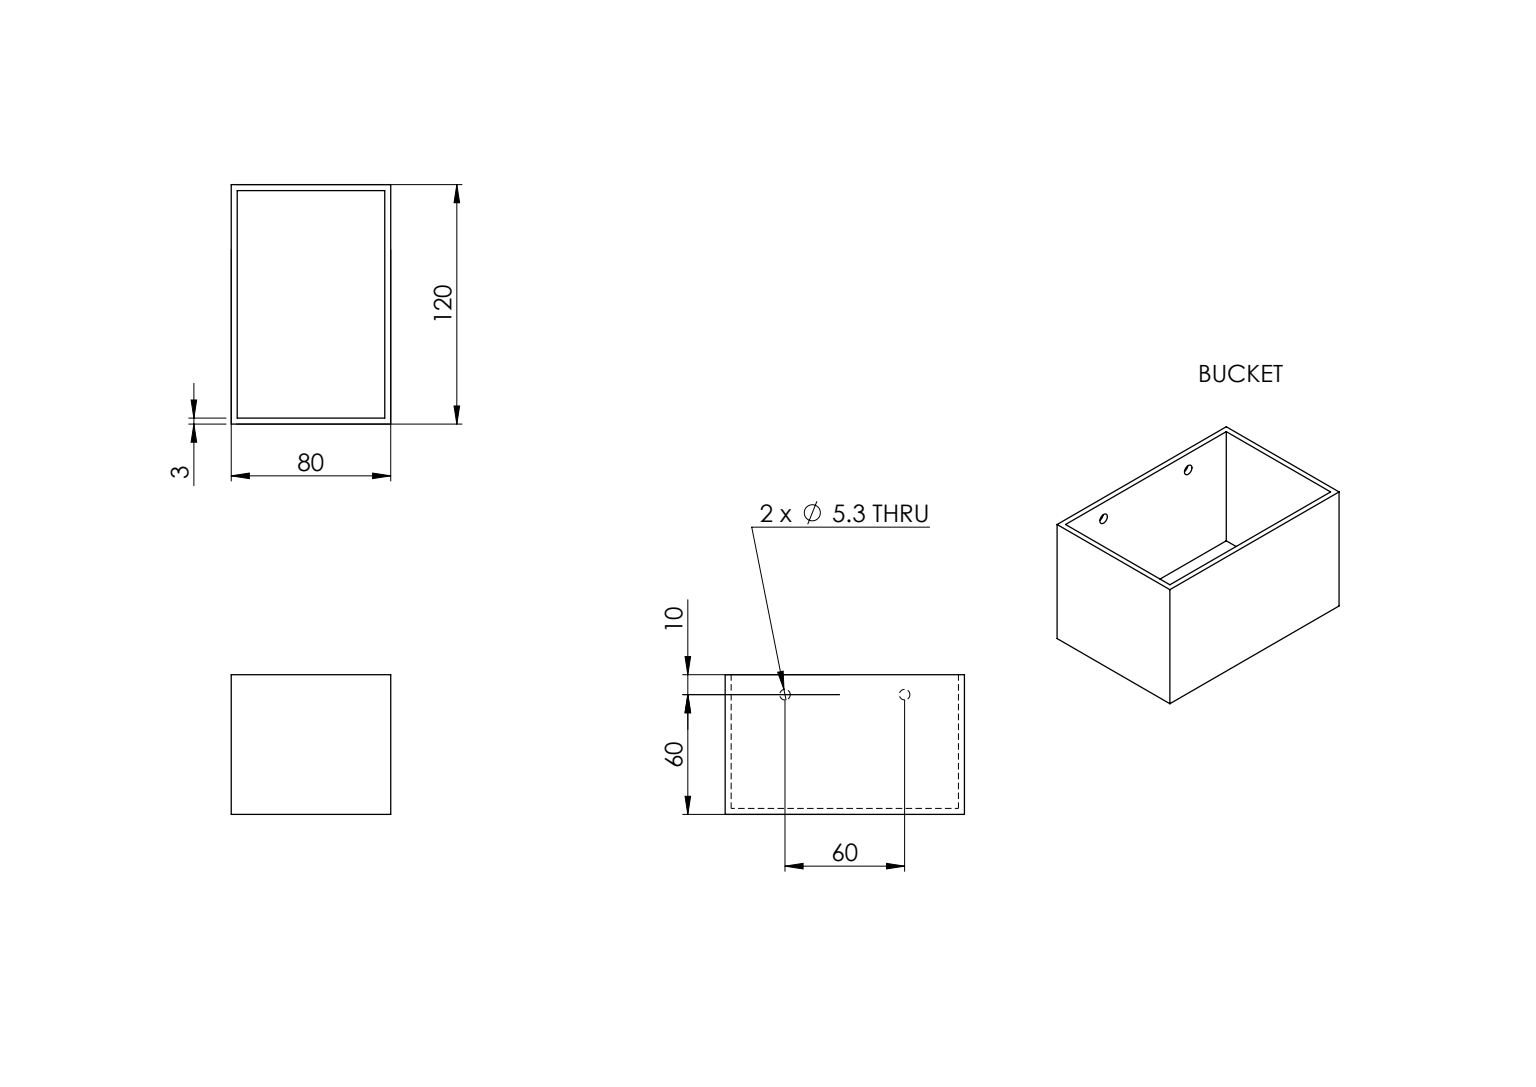
ISO-10303-21;
HEADER;
FILE_DESCRIPTION (('STEP AP214'),
    '1' );
FILE_NAME ('bucket.step',
    '2026-10-31T03:46:07',
    ( '' ),
    ( '' ),
    'SwSTEP 2.0',
    'SolidWorks 2026',
    '' );
FILE_SCHEMA (( 'AUTOMOTIVE_DESIGN' ));
ENDSEC;

DATA;
#88=ADVANCED_FACE ( 'NONE', ( #16201 ), #18340, .T. ) ;
#110=SHAPE_DEFINITION_REPRESENTATION ( #7281, #4815 ) ;
#112=DIRECTION ( 'NONE',  ( 1.302872740555339390E-32, -4.694093751100962712E-16, 1.000000000000000000 ) ) ;
#206=ORIENTED_EDGE ( 'NONE', *, *, #14942, .F. ) ;
#227=VECTOR ( 'NONE', #939, 1000.000000000000000 ) ;
#320=EDGE_CURVE ( 'NONE', #20633, #11416, #17854, .T. ) ;
#350=AXIS2_PLACEMENT_3D ( 'NONE', #4294, #21542, #12071 ) ;
#400=ORIENTED_EDGE ( 'NONE', *, *, #3148, .F. ) ;
#413=AXIS2_PLACEMENT_3D ( 'NONE', #9639, #22415, #8058 ) ;
#456=PLANE ( 'NONE',  #413 ) ;
#469=UNCERTAINTY_MEASURE_WITH_UNIT (LENGTH_MEASURE( 1.000000000000000082E-05 ), #4859, 'distance_accuracy_value', 'NONE');
#495=FACE_OUTER_BOUND ( 'NONE', #9438, .T. ) ;
#523=DIRECTION ( 'NONE',  ( -1.000000000000000000, -2.775557561562891351E-17, -0.000000000000000000 ) ) ;
#544=ADVANCED_FACE ( 'NONE', ( #5876 ), #11344, .F. ) ;
#592=DIRECTION ( 'NONE',  ( -2.775557561562891351E-17, 1.000000000000000000, -1.850371707708594366E-15 ) ) ;
#605=CARTESIAN_POINT ( 'NONE',  ( 158.0000000000000284, -500.0000000000000000, 32.64999999999999858 ) ) ;
#610=DIRECTION ( 'NONE',  ( -1.000000000000000000, -2.775557561562891351E-17, -0.000000000000000000 ) ) ;
#638=CARTESIAN_POINT ( 'NONE',  ( 158.0000000000000284, -490.0000000000001137, -56.99999999999996447 ) ) ;
#651=CARTESIAN_POINT ( 'NONE',  ( 235.0000000000000284, 6.522560269672795464E-15, 0.000000000000000000 ) ) ;
#718=LINE ( 'NONE', #21363, #15052 ) ;
#728=CARTESIAN_POINT ( 'NONE',  ( 235.0000000000000284, -499.9999999999999432, -59.99999999999997868 ) ) ;
#812=DIRECTION ( 'NONE',  ( 0.000000000000000000, 0.000000000000000000, -1.000000000000000000 ) ) ;
#827=PLANE ( 'NONE',  #4915 ) ;
#859=DIRECTION ( 'NONE',  ( -1.000000000000000000, -2.775557561562891351E-17, 0.000000000000000000 ) ) ;
#896=MECHANICAL_DESIGN_GEOMETRIC_PRESENTATION_REPRESENTATION('',(#6700),#10991);
#918=DIRECTION ( 'NONE',  ( 1.000000000000000000, -0.000000000000000000, -0.000000000000000000 ) ) ;
#939=DIRECTION ( 'NONE',  ( 1.000000000000000000, -0.000000000000000000, -0.000000000000000000 ) ) ;
#973=ORIENTED_EDGE ( 'NONE', *, *, #1611, .T. ) ;
#1108=( NAMED_UNIT ( * ) SI_UNIT ( $, .STERADIAN. ) SOLID_ANGLE_UNIT ( ) );
#1140=AXIS2_PLACEMENT_3D ( 'NONE', #651, #11317, #18625 ) ;
#1188=EDGE_CURVE ( 'NONE', #12219, #19824, #2031, .T. ) ;
#1230=ORIENTED_EDGE ( 'NONE', *, *, #6445, .T. ) ;
#1269=EDGE_LOOP ( 'NONE', ( #15243, #18785, #1846, #6416 ) ) ;
#1280=VECTOR ( 'NONE', #12258, 1000.000000000000000 ) ;
#1383=VECTOR ( 'NONE', #18125, 1000.000000000000000 ) ;
#1452=VECTOR ( 'NONE', #1843, 1000.000000000000000 ) ;
#1510=AXIS2_PLACEMENT_3D ( 'NONE', #7279, #14677, #17066 ) ;
#1611=EDGE_CURVE ( 'NONE', #21138, #9885, #12704, .T. ) ;
#1615=CARTESIAN_POINT ( 'NONE',  ( 235.0000000000000284, -557.0000000000000000, -60.00000000000000711 ) ) ;
#1694=DIRECTION ( 'NONE',  ( 0.000000000000000000, -1.000000000000000000, 0.000000000000000000 ) ) ;
#1739=DIRECTION ( 'NONE',  ( 1.000000000000000000, -0.000000000000000000, -0.000000000000000000 ) ) ;
#1843=DIRECTION ( 'NONE',  ( 5.135813185032629306E-32, -1.850371707708594366E-15, -1.000000000000000000 ) ) ;
#1846=ORIENTED_EDGE ( 'NONE', *, *, #10977, .T. ) ;
#1897=EDGE_CURVE ( 'NONE', #17629, #8807, #23245, .T. ) ;
#1906=( GEOMETRIC_REPRESENTATION_CONTEXT ( 3 ) GLOBAL_UNCERTAINTY_ASSIGNED_CONTEXT ( ( #469 ) ) GLOBAL_UNIT_ASSIGNED_CONTEXT ( ( #4859, #14311, #1108 ) ) REPRESENTATION_CONTEXT ( 'NONE', 'WORKASPACE' ) );
#1913=LINE ( 'NONE', #14861, #19155 ) ;
#1918=EDGE_LOOP ( 'NONE', ( #7609, #8535, #973, #13571 ) ) ;
#1919=DIRECTION ( 'NONE',  ( 1.000000000000000000, 2.775557561562891351E-17, 0.000000000000000000 ) ) ;
#1934=EDGE_CURVE ( 'NONE', #17283, #16779, #5492, .T. ) ;
#1935=( NAMED_UNIT ( * ) PLANE_ANGLE_UNIT ( ) SI_UNIT ( $, .RADIAN. ) );
#2031=LINE ( 'NONE', #10783, #1383 ) ;
#2092=VECTOR ( 'NONE', #1739, 1000.000000000000000 ) ;
#2117=CIRCLE ( 'NONE', #16041, 2.650000000000041211 ) ;
#2154=ORIENTED_EDGE ( 'NONE', *, *, #13234, .T. ) ;
#2162=CARTESIAN_POINT ( 'NONE',  ( 155.0000000000000284, -500.0000000000000000, -32.64999999999995595 ) ) ;
#2173=CARTESIAN_POINT ( 'NONE',  ( 232.0000000000000284, -489.9999999999998863, 57.00000000000002132 ) ) ;
#2238=FACE_BOUND ( 'NONE', #22062, .T. ) ;
#2261=CIRCLE ( 'NONE', #350, 2.650000000000041211 ) ;
#2336=LINE ( 'NONE', #9962, #8477 ) ;
#2369=FACE_BOUND ( 'NONE', #18057, .T. ) ;
#2408=CARTESIAN_POINT ( 'NONE',  ( 158.0000000000000284, -500.0000000000000000, 30.00000000000001421 ) ) ;
#2488=FACE_OUTER_BOUND ( 'NONE', #11813, .T. ) ;
#2529=LINE ( 'NONE', #6033, #13147 ) ;
#2531=LINE ( 'NONE', #18818, #20422 ) ;
#2557=LINE ( 'NONE', #15384, #17979 ) ;
#2682=CARTESIAN_POINT ( 'NONE',  ( 235.0000000000000284, -557.0000000000000000, 56.99999999999998579 ) ) ;
#2843=FACE_OUTER_BOUND ( 'NONE', #1269, .T. ) ;
#2859=CARTESIAN_POINT ( 'NONE',  ( 155.0000000000000284, -490.0000000000001137, -60.00000000000000000 ) ) ;
#2864=CARTESIAN_POINT ( 'NONE',  ( 155.0000000000000568, -560.0000000000000000, 59.99999999999999289 ) ) ;
#2871=ORIENTED_EDGE ( 'NONE', *, *, #16274, .T. ) ;
#2880=FACE_BOUND ( 'NONE', #9684, .T. ) ;
#2981=CIRCLE ( 'NONE', #18802, 2.650000000000041211 ) ;
#2987=CIRCLE ( 'NONE', #12307, 2.649999999999985700 ) ;
#3030=( LENGTH_UNIT ( ) NAMED_UNIT ( * ) SI_UNIT ( .MILLI., .METRE. ) );
#3126=ORIENTED_EDGE ( 'NONE', *, *, #9156, .T. ) ;
#3148=EDGE_CURVE ( 'NONE', #16779, #14572, #23143, .T. ) ;
#3229=ADVANCED_BREP_SHAPE_REPRESENTATION ( '', ( #12677, #11210 ), #1906 ) ;
#3271=SHAPE_REPRESENTATION_RELATIONSHIP ( 'NONE' , 'NONE' ,  #4815, #3229 ) ;
#3340=ORIENTED_EDGE ( 'NONE', *, *, #21968, .F. ) ;
#3470=AXIS2_PLACEMENT_3D ( 'NONE', #2408, #6034, #11754 ) ;
#3553=LINE ( 'NONE', #18530, #2092 ) ;
#3686=EDGE_LOOP ( 'NONE', ( #14401, #21703, #12674, #4879 ) ) ;
#3699=CARTESIAN_POINT ( 'NONE',  ( 235.0000000000000284, -489.9999999999998863, 60.00000000000000000 ) ) ;
#3706=PRODUCT_CONTEXT ( 'NONE', #18458, 'mechanical' ) ;
#3769=DIRECTION ( 'NONE',  ( 1.000000000000000000, 0.000000000000000000, 0.000000000000000000 ) ) ;
#3804=ORIENTED_EDGE ( 'NONE', *, *, #12596, .F. ) ;
#3892=ORIENTED_EDGE ( 'NONE', *, *, #14111, .T. ) ;
#4033=DIRECTION ( 'NONE',  ( 1.000000000000000000, -0.000000000000000000, -0.000000000000000000 ) ) ;
#4050=DIRECTION ( 'NONE',  ( 1.302872740555339390E-32, -4.694093751100962712E-16, 1.000000000000000000 ) ) ;
#4149=EDGE_CURVE ( 'NONE', #21138, #22960, #6894, .T. ) ;
#4276=LINE ( 'NONE', #11429, #16601 ) ;
#4294=CARTESIAN_POINT ( 'NONE',  ( 155.0000000000000284, -500.0000000000000000, -29.99999999999997158 ) ) ;
#4421=VERTEX_POINT ( 'NONE', #7599 ) ;
#4469=EDGE_LOOP ( 'NONE', ( #4649, #11714, #18366, #18198 ) ) ;
#4526=FACE_OUTER_BOUND ( 'NONE', #4469, .T. ) ;
#4580=CARTESIAN_POINT ( 'NONE',  ( 155.0000000000000284, -500.0000000000000000, 30.00000000000001421 ) ) ;
#4589=EDGE_CURVE ( 'NONE', #21635, #20633, #2117, .T. ) ;
#4639=VECTOR ( 'NONE', #12672, 1000.000000000000000 ) ;
#4649=ORIENTED_EDGE ( 'NONE', *, *, #1934, .F. ) ;
#4712=ORIENTED_EDGE ( 'NONE', *, *, #13940, .T. ) ;
#4760=VERTEX_POINT ( 'NONE', #18888 ) ;
#4815=SHAPE_REPRESENTATION ( 'bucket', ( #11210 ), #1906 ) ;
#4816=ORIENTED_EDGE ( 'NONE', *, *, #320, .T. ) ;
#4822=DIRECTION ( 'NONE',  ( -1.000000000000000000, -2.775557561562891351E-17, 0.000000000000000000 ) ) ;
#4837=CLOSED_SHELL ( 'NONE', ( #20163, #5626, #8681, #22263, #88, #8337, #10668, #10191, #544, #13232, #22991, #23443, #8416, #18584, #14331 ) ) ;
#4857=ORIENTED_EDGE ( 'NONE', *, *, #13940, .F. ) ;
#4859=( LENGTH_UNIT ( ) NAMED_UNIT ( * ) SI_UNIT ( .MILLI., .METRE. ) );
#4879=ORIENTED_EDGE ( 'NONE', *, *, #5633, .T. ) ;
#4894=DIRECTION ( 'NONE',  ( -1.000000000000000000, -2.775557561562891351E-17, -0.000000000000000000 ) ) ;
#4915=AXIS2_PLACEMENT_3D ( 'NONE', #17135, #592, #7956 ) ;
#4947=ORIENTED_EDGE ( 'NONE', *, *, #21843, .F. ) ;
#4982=EDGE_LOOP ( 'NONE', ( #11522, #8071, #3340, #14686 ) ) ;
#5015=( GEOMETRIC_REPRESENTATION_CONTEXT ( 3 ) GLOBAL_UNCERTAINTY_ASSIGNED_CONTEXT ( ( #22660 ) ) GLOBAL_UNIT_ASSIGNED_CONTEXT ( ( #3030, #21289, #23324 ) ) REPRESENTATION_CONTEXT ( 'NONE', 'WORKASPACE' ) );
#5102=FILL_AREA_STYLE ('',( #10446 ) ) ;
#5178=CARTESIAN_POINT ( 'NONE',  ( 235.0000000000000284, -499.9999999999998863, 60.00000000000002132 ) ) ;
#5286=EDGE_CURVE ( 'NONE', #17629, #7103, #2557, .T. ) ;
#5437=DIRECTION ( 'NONE',  ( 0.000000000000000000, 0.000000000000000000, 1.000000000000000000 ) ) ;
#5492=LINE ( 'NONE', #8910, #19581 ) ;
#5533=ORIENTED_EDGE ( 'NONE', *, *, #9323, .F. ) ;
#5601=DIRECTION ( 'NONE',  ( 0.000000000000000000, -1.000000000000000000, 0.000000000000000000 ) ) ;
#5626=ADVANCED_FACE ( 'NONE', ( #495 ), #20759, .F. ) ;
#5633=EDGE_CURVE ( 'NONE', #8807, #17283, #2531, .T. ) ;
#5642=DIRECTION ( 'NONE',  ( 0.000000000000000000, -1.000000000000000000, -4.694093751100962712E-16 ) ) ;
#5720=VECTOR ( 'NONE', #17826, 1000.000000000000000 ) ;
#5791=VECTOR ( 'NONE', #13227, 1000.000000000000000 ) ;
#5876=FACE_OUTER_BOUND ( 'NONE', #23483, .T. ) ;
#5893=CARTESIAN_POINT ( 'NONE',  ( 235.0000000000000284, -499.9999999999999432, -56.99999999999997158 ) ) ;
#5900=PRODUCT_DEFINITION_CONTEXT ( 'detailed design', #23255, 'design' ) ;
#5904=ORIENTED_EDGE ( 'NONE', *, *, #12596, .T. ) ;
#5980=PLANE ( 'NONE',  #22662 ) ;
#6033=CARTESIAN_POINT ( 'NONE',  ( 232.0000000000000284, -490.0000000000000000, 9.066821367772113093E-13 ) ) ;
#6034=DIRECTION ( 'NONE',  ( 1.000000000000000000, -0.000000000000000000, -0.000000000000000000 ) ) ;
#6158=MECHANICAL_DESIGN_GEOMETRIC_PRESENTATION_REPRESENTATION('',(#6557),#5015);
#6225=ORIENTED_EDGE ( 'NONE', *, *, #10037, .F. ) ;
#6275=ORIENTED_EDGE ( 'NONE', *, *, #1611, .F. ) ;
#6345=VERTEX_POINT ( 'NONE', #7187 ) ;
#6363=DIRECTION ( 'NONE',  ( 0.000000000000000000, 0.000000000000000000, -1.000000000000000000 ) ) ;
#6380=FACE_BOUND ( 'NONE', #12034, .T. ) ;
#6416=ORIENTED_EDGE ( 'NONE', *, *, #14942, .T. ) ;
#6437=ORIENTED_EDGE ( 'NONE', *, *, #19331, .T. ) ;
#6445=EDGE_CURVE ( 'NONE', #10663, #11416, #18841, .T. ) ;
#6530=ORIENTED_EDGE ( 'NONE', *, *, #16274, .F. ) ;
#6557=STYLED_ITEM ( 'NONE', ( #19569 ), #3229 ) ;
#6627=LINE ( 'NONE', #14023, #16227 ) ;
#6684=VECTOR ( 'NONE', #10622, 1000.000000000000000 ) ;
#6700=STYLED_ITEM('',(#23913),#12677);
#6756=VECTOR ( 'NONE', #859, 1000.000000000000000 ) ;
#6816=LINE ( 'NONE', #16006, #8271 ) ;
#6894=LINE ( 'NONE', #2682, #6756 ) ;
#6943=DIRECTION ( 'NONE',  ( 1.000000000000000000, -0.000000000000000000, -0.000000000000000000 ) ) ;
#6952=CARTESIAN_POINT ( 'NONE',  ( 155.0000000000000284, -500.0000000000000000, -29.99999999999997158 ) ) ;
#6962=DIRECTION ( 'NONE',  ( -2.775557561562891351E-17, 1.000000000000000000, 4.694093751100962712E-16 ) ) ;
#6997=DIRECTION ( 'NONE',  ( -2.775557561562891351E-17, 1.000000000000000000, -2.081668171172166936E-15 ) ) ;
#7083=CARTESIAN_POINT ( 'NONE',  ( 158.0000000000000284, -500.0000000000000000, 27.35000000000002629 ) ) ;
#7103=VERTEX_POINT ( 'NONE', #10126 ) ;
#7162=DIRECTION ( 'NONE',  ( 2.775557561562891351E-17, -1.000000000000000000, 0.000000000000000000 ) ) ;
#7187=CARTESIAN_POINT ( 'NONE',  ( 235.0000000000000284, -489.9999999999998863, 60.00000000000000000 ) ) ;
#7279=CARTESIAN_POINT ( 'NONE',  ( 158.0000000000000284, -500.0000000000000000, -29.99999999999997158 ) ) ;
#7281=PRODUCT_DEFINITION_SHAPE ( 'NONE', 'NONE',  #7979 ) ;
#7382=ORIENTED_EDGE ( 'NONE', *, *, #7713, .F. ) ;
#7431=CARTESIAN_POINT ( 'NONE',  ( 155.0000000000000284, -500.0000000000000000, -27.34999999999998721 ) ) ;
#7435=CARTESIAN_POINT ( 'NONE',  ( 235.0000000000000284, -557.0000000000000000, -57.00000000000000000 ) ) ;
#7469=DIRECTION ( 'NONE',  ( 2.775557561562891351E-17, -1.000000000000000000, 0.000000000000000000 ) ) ;
#7599=CARTESIAN_POINT ( 'NONE',  ( 158.0000000000000284, -500.0000000000000000, -32.64999999999995595 ) ) ;
#7609=ORIENTED_EDGE ( 'NONE', *, *, #14111, .F. ) ;
#7678=DIRECTION ( 'NONE',  ( -0.000000000000000000, 0.000000000000000000, 1.000000000000000000 ) ) ;
#7713=EDGE_CURVE ( 'NONE', #21635, #10663, #16284, .T. ) ;
#7749=CARTESIAN_POINT ( 'NONE',  ( 155.0000000000000284, -500.0000000000000000, 30.00000000000001421 ) ) ;
#7892=EDGE_LOOP ( 'NONE', ( #18868, #4712, #10129, #1230 ) ) ;
#7898=PLANE ( 'NONE',  #1140 ) ;
#7917=LINE ( 'NONE', #7435, #8635 ) ;
#7956=DIRECTION ( 'NONE',  ( 0.000000000000000000, 1.850371707708594366E-15, 1.000000000000000000 ) ) ;
#7979=PRODUCT_DEFINITION ( 'UNKNOWN', '', #10444, #5900 ) ;
#7985=AXIS2_PLACEMENT_3D ( 'NONE', #728, #16198, #15848 ) ;
#8020=FACE_OUTER_BOUND ( 'NONE', #4982, .T. ) ;
#8040=DIRECTION ( 'NONE',  ( 0.000000000000000000, -1.000000000000000000, -4.694093751100962712E-16 ) ) ;
#8049=AXIS2_PLACEMENT_3D ( 'NONE', #5893, #112, #16766 ) ;
#8058=DIRECTION ( 'NONE',  ( -0.000000000000000000, 0.000000000000000000, 1.000000000000000000 ) ) ;
#8071=ORIENTED_EDGE ( 'NONE', *, *, #9329, .F. ) ;
#8116=EDGE_LOOP ( 'NONE', ( #13521, #17499, #3892, #5904 ) ) ;
#8197=CARTESIAN_POINT ( 'NONE',  ( 158.0000000000000284, -500.0000000000000000, -29.99999999999997158 ) ) ;
#8241=ORIENTED_EDGE ( 'NONE', *, *, #12011, .F. ) ;
#8271=VECTOR ( 'NONE', #21547, 1000.000000000000000 ) ;
#8326=DIRECTION ( 'NONE',  ( -1.000000000000000000, -2.775557561562891351E-17, 0.000000000000000000 ) ) ;
#8337=ADVANCED_FACE ( 'NONE', ( #19317 ), #17285, .F. ) ;
#8416=ADVANCED_FACE ( 'NONE', ( #2880, #10657, #12375 ), #10539, .F. ) ;
#8474=VERTEX_POINT ( 'NONE', #12954 ) ;
#8477=VECTOR ( 'NONE', #17078, 1000.000000000000000 ) ;
#8532=LINE ( 'NONE', #8641, #18051 ) ;
#8535=ORIENTED_EDGE ( 'NONE', *, *, #10655, .T. ) ;
#8549=EDGE_CURVE ( 'NONE', #7103, #17283, #1913, .T. ) ;
#8550=ORIENTED_EDGE ( 'NONE', *, *, #22469, .T. ) ;
#8635=VECTOR ( 'NONE', #15182, 1000.000000000000000 ) ;
#8641=CARTESIAN_POINT ( 'NONE',  ( 235.0000000000000284, -490.0000000000001137, -60.00000000000000000 ) ) ;
#8681=ADVANCED_FACE ( 'NONE', ( #22802, #6380 ), #827, .T. ) ;
#8730=SURFACE_STYLE_USAGE ( .BOTH. , #14069 ) ;
#8762=CARTESIAN_POINT ( 'NONE',  ( 158.0000000000000284, 3.114171532854473382E-14, -56.99999999999973710 ) ) ;
#8795=VECTOR ( 'NONE', #20249, 1000.000000000000000 ) ;
#8807=VERTEX_POINT ( 'NONE', #17598 ) ;
#8889=PLANE ( 'NONE',  #15229 ) ;
#8910=CARTESIAN_POINT ( 'NONE',  ( 155.0000000000000284, -500.0000000000000000, 60.00000000000002132 ) ) ;
#9156=EDGE_CURVE ( 'NONE', #4760, #14572, #8532, .T. ) ;
#9222=AXIS2_PLACEMENT_3D ( 'NONE', #14709, #9383, #7678 ) ;
#9311=ORIENTED_EDGE ( 'NONE', *, *, #9852, .F. ) ;
#9323=EDGE_CURVE ( 'NONE', #12219, #20656, #2981, .T. ) ;
#9329=EDGE_CURVE ( 'NONE', #6345, #4760, #10845, .T. ) ;
#9383=DIRECTION ( 'NONE',  ( -1.000000000000000000, -2.775557561562891351E-17, 0.000000000000000000 ) ) ;
#9409=FACE_OUTER_BOUND ( 'NONE', #8116, .T. ) ;
#9433=( NAMED_UNIT ( * ) SI_UNIT ( $, .STERADIAN. ) SOLID_ANGLE_UNIT ( ) );
#9438=EDGE_LOOP ( 'NONE', ( #19154, #4816, #8550, #7382 ) ) ;
#9458=ORIENTED_EDGE ( 'NONE', *, *, #10655, .F. ) ;
#9473=CARTESIAN_POINT ( 'NONE',  ( 0.000000000000000000, 0.000000000000000000, 0.000000000000000000 ) ) ;
#9499=CARTESIAN_POINT ( 'NONE',  ( 158.0000000000000284, -500.0000000000000000, 30.00000000000001421 ) ) ;
#9639=CARTESIAN_POINT ( 'NONE',  ( 155.0000000000000284, 4.302114220422482383E-15, 0.000000000000000000 ) ) ;
#9684=EDGE_LOOP ( 'NONE', ( #206, #8241 ) ) ;
#9759=ORIENTED_EDGE ( 'NONE', *, *, #9852, .T. ) ;
#9852=EDGE_CURVE ( 'NONE', #18604, #20252, #15009, .T. ) ;
#9885=VERTEX_POINT ( 'NONE', #2173 ) ;
#9915=FACE_OUTER_BOUND ( 'NONE', #1918, .T. ) ;
#9962=CARTESIAN_POINT ( 'NONE',  ( 232.0000000000000568, -557.0000000000000000, 0.000000000000000000 ) ) ;
#10035=AXIS2_PLACEMENT_3D ( 'NONE', #15320, #918, #812 ) ;
#10037=EDGE_CURVE ( 'NONE', #7103, #14572, #6627, .T. ) ;
#10126=CARTESIAN_POINT ( 'NONE',  ( 155.0000000000000568, -560.0000000000000000, -60.00000000000000711 ) ) ;
#10129=ORIENTED_EDGE ( 'NONE', *, *, #7713, .T. ) ;
#10130=CARTESIAN_POINT ( 'NONE',  ( 158.0000000000000284, -489.9999999999998863, 57.00000000000002132 ) ) ;
#10191=ADVANCED_FACE ( 'NONE', ( #2238, #2369, #2488 ), #456, .T. ) ;
#10207=CIRCLE ( 'NONE', #18267, 2.649999999999985700 ) ;
#10216=DIRECTION ( 'NONE',  ( 0.000000000000000000, 0.000000000000000000, -1.000000000000000000 ) ) ;
#10250=VECTOR ( 'NONE', #10755, 1000.000000000000000 ) ;
#10274=DIRECTION ( 'NONE',  ( 0.000000000000000000, -1.000000000000000000, 0.000000000000000000 ) ) ;
#10285=CARTESIAN_POINT ( 'NONE',  ( 158.0000000000000284, 4.385380947269369124E-15, 0.000000000000000000 ) ) ;
#10308=VERTEX_POINT ( 'NONE', #22884 ) ;
#10343=ORIENTED_EDGE ( 'NONE', *, *, #1188, .T. ) ;
#10444=PRODUCT_DEFINITION_FORMATION_WITH_SPECIFIED_SOURCE ( 'ANY', '', #23666, .NOT_KNOWN. ) ;
#10446=FILL_AREA_STYLE_COLOUR ( '', #15835 ) ;
#10460=ORIENTED_EDGE ( 'NONE', *, *, #20025, .T. ) ;
#10539=PLANE ( 'NONE',  #14543 ) ;
#10622=DIRECTION ( 'NONE',  ( 1.000000000000000000, -0.000000000000000000, -0.000000000000000000 ) ) ;
#10655=EDGE_CURVE ( 'NONE', #8474, #21138, #2336, .T. ) ;
#10657=FACE_BOUND ( 'NONE', #23043, .T. ) ;
#10663=VERTEX_POINT ( 'NONE', #18743 ) ;
#10668=ADVANCED_FACE ( 'NONE', ( #8020 ), #7898, .F. ) ;
#10755=DIRECTION ( 'NONE',  ( -2.775557561562891351E-17, 1.000000000000000000, 4.694093751100962712E-16 ) ) ;
#10783=CARTESIAN_POINT ( 'NONE',  ( 158.0000000000000284, -500.0000000000000000, -27.34999999999998721 ) ) ;
#10845=LINE ( 'NONE', #14556, #1452 ) ;
#10946=DIRECTION ( 'NONE',  ( 1.000000000000000000, 2.775557561562891351E-17, 0.000000000000000000 ) ) ;
#10958=LINE ( 'NONE', #22029, #21899 ) ;
#10977=EDGE_CURVE ( 'NONE', #20656, #4421, #3553, .T. ) ;
#10991=( GEOMETRIC_REPRESENTATION_CONTEXT ( 3 ) GLOBAL_UNCERTAINTY_ASSIGNED_CONTEXT ( ( #11901 ) ) GLOBAL_UNIT_ASSIGNED_CONTEXT ( ( #18586, #1935, #9433 ) ) REPRESENTATION_CONTEXT ( 'NONE', 'WORKASPACE' ) );
#10996=CARTESIAN_POINT ( 'NONE',  ( 232.0000000000000284, -2.031704083844970052E-14, 57.00000000000024869 ) ) ;
#11210=AXIS2_PLACEMENT_3D ( 'NONE', #9473, #14914, #3769 ) ;
#11317=DIRECTION ( 'NONE',  ( -1.000000000000000000, -2.775557561562891351E-17, 0.000000000000000000 ) ) ;
#11344=PLANE ( 'NONE',  #12193 ) ;
#11416=VERTEX_POINT ( 'NONE', #605 ) ;
#11429=CARTESIAN_POINT ( 'NONE',  ( 235.0000000000000284, -500.0000000000001137, -59.99999999999997868 ) ) ;
#11456=DIRECTION ( 'NONE',  ( 0.000000000000000000, 0.000000000000000000, -1.000000000000000000 ) ) ;
#11490=ORIENTED_EDGE ( 'NONE', *, *, #4589, .F. ) ;
#11522=ORIENTED_EDGE ( 'NONE', *, *, #15278, .T. ) ;
#11705=ORIENTED_EDGE ( 'NONE', *, *, #13234, .F. ) ;
#11714=ORIENTED_EDGE ( 'NONE', *, *, #5633, .F. ) ;
#11754=DIRECTION ( 'NONE',  ( 0.000000000000000000, 0.000000000000000000, -1.000000000000000000 ) ) ;
#11813=EDGE_LOOP ( 'NONE', ( #17897, #6225, #19204, #15871 ) ) ;
#11901=UNCERTAINTY_MEASURE_WITH_UNIT (LENGTH_MEASURE( 1.000000000000000082E-05 ), #18586, 'distance_accuracy_value', 'NONE');
#11968=CYLINDRICAL_SURFACE ( 'NONE', #10035, 2.649999999999985700 ) ;
#12011=EDGE_CURVE ( 'NONE', #19824, #4421, #10207, .T. ) ;
#12034=EDGE_LOOP ( 'NONE', ( #6437, #9759, #3804, #23410 ) ) ;
#12071=DIRECTION ( 'NONE',  ( 0.000000000000000000, -1.000000000000000000, 0.000000000000000000 ) ) ;
#12091=EDGE_LOOP ( 'NONE', ( #400, #4947, #17257, #3126 ) ) ;
#12129=EDGE_LOOP ( 'NONE', ( #2154, #22010, #9458, #17968 ) ) ;
#12193=AXIS2_PLACEMENT_3D ( 'NONE', #16751, #4050, #5642 ) ;
#12219=VERTEX_POINT ( 'NONE', #7431 ) ;
#12258=DIRECTION ( 'NONE',  ( -1.000000000000000000, -2.775557561562891351E-17, 0.000000000000000000 ) ) ;
#12293=CARTESIAN_POINT ( 'NONE',  ( 158.0000000000000284, -500.0000000000000000, 30.00000000000001421 ) ) ;
#12307=AXIS2_PLACEMENT_3D ( 'NONE', #12293, #6943, #10216 ) ;
#12375=FACE_OUTER_BOUND ( 'NONE', #22943, .T. ) ;
#12596=EDGE_CURVE ( 'NONE', #14788, #20252, #17641, .T. ) ;
#12672=DIRECTION ( 'NONE',  ( 5.135813185032629306E-32, -1.850371707708594366E-15, -1.000000000000000000 ) ) ;
#12674=ORIENTED_EDGE ( 'NONE', *, *, #1897, .T. ) ;
#12677=MANIFOLD_SOLID_BREP ( 'M5 Clearance Hole1', #4837 ) ;
#12704=LINE ( 'NONE', #10996, #10250 ) ;
#12787=LINE ( 'NONE', #8762, #13705 ) ;
#12912=ORIENTED_EDGE ( 'NONE', *, *, #5286, .T. ) ;
#12954=CARTESIAN_POINT ( 'NONE',  ( 232.0000000000000568, -557.0000000000000000, -57.00000000000000000 ) ) ;
#12955=EDGE_CURVE ( 'NONE', #8474, #10308, #7917, .T. ) ;
#12976=CARTESIAN_POINT ( 'NONE',  ( 155.0000000000000284, -500.0000000000000000, 27.35000000000002629 ) ) ;
#13147=VECTOR ( 'NONE', #21128, 1000.000000000000000 ) ;
#13227=DIRECTION ( 'NONE',  ( 5.135813185032629306E-32, -1.850371707708594366E-15, -1.000000000000000000 ) ) ;
#13232=ADVANCED_FACE ( 'NONE', ( #19962 ), #8889, .F. ) ;
#13234=EDGE_CURVE ( 'NONE', #10308, #22960, #6816, .T. ) ;
#13297=EDGE_CURVE ( 'NONE', #10308, #20252, #12787, .T. ) ;
#13375=CARTESIAN_POINT ( 'NONE',  ( 235.0000000000000284, -560.0000000000000000, -60.00000000000000711 ) ) ;
#13389=CARTESIAN_POINT ( 'NONE',  ( 235.0000000000000284, -500.0000000000000000, 60.00000000000002132 ) ) ;
#13419=PLANE ( 'NONE',  #8049 ) ;
#13521=ORIENTED_EDGE ( 'NONE', *, *, #13297, .F. ) ;
#13524=DIRECTION ( 'NONE',  ( 1.302872740555339390E-32, -4.694093751100962712E-16, 1.000000000000000000 ) ) ;
#13571=ORIENTED_EDGE ( 'NONE', *, *, #19305, .T. ) ;
#13705=VECTOR ( 'NONE', #16122, 1000.000000000000000 ) ;
#13708=AXIS2_PLACEMENT_3D ( 'NONE', #14510, #7469, #1919 ) ;
#13769=CARTESIAN_POINT ( 'NONE',  ( 235.0000000000000284, -560.0000000000000000, -60.00000000000000711 ) ) ;
#13940=EDGE_CURVE ( 'NONE', #20633, #21635, #22698, .T. ) ;
#14023=CARTESIAN_POINT ( 'NONE',  ( 155.0000000000000284, -499.9999999999999432, -59.99999999999997868 ) ) ;
#14069=SURFACE_SIDE_STYLE ('',( #19339 ) ) ;
#14111=EDGE_CURVE ( 'NONE', #8474, #14788, #20487, .T. ) ;
#14137=DIRECTION ( 'NONE',  ( -2.775557561562891351E-17, 1.000000000000000000, 4.694093751100962712E-16 ) ) ;
#14236=FACE_OUTER_BOUND ( 'NONE', #7892, .T. ) ;
#14311=( NAMED_UNIT ( * ) PLANE_ANGLE_UNIT ( ) SI_UNIT ( $, .RADIAN. ) );
#14331=ADVANCED_FACE ( 'NONE', ( #2843 ), #11968, .F. ) ;
#14349=DIRECTION ( 'NONE',  ( -2.775557561562891351E-17, 1.000000000000000000, 4.694093751100962712E-16 ) ) ;
#14401=ORIENTED_EDGE ( 'NONE', *, *, #8549, .F. ) ;
#14510=CARTESIAN_POINT ( 'NONE',  ( 235.0000000000000284, -560.0000000000000000, -60.00000000000000711 ) ) ;
#14543=AXIS2_PLACEMENT_3D ( 'NONE', #10285, #17873, #21735 ) ;
#14556=CARTESIAN_POINT ( 'NONE',  ( 235.0000000000000284, -489.9999999999998863, 60.00000000000000000 ) ) ;
#14572=VERTEX_POINT ( 'NONE', #2859 ) ;
#14631=AXIS2_PLACEMENT_3D ( 'NONE', #9499, #4033, #16850 ) ;
#14637=AXIS2_PLACEMENT_3D ( 'NONE', #7749, #22458, #1694 ) ;
#14677=DIRECTION ( 'NONE',  ( 1.000000000000000000, -0.000000000000000000, -0.000000000000000000 ) ) ;
#14686=ORIENTED_EDGE ( 'NONE', *, *, #1897, .F. ) ;
#14709=CARTESIAN_POINT ( 'NONE',  ( 232.0000000000000284, 6.439293542825908723E-15, 0.000000000000000000 ) ) ;
#14729=LINE ( 'NONE', #3699, #8795 ) ;
#14788=VERTEX_POINT ( 'NONE', #23741 ) ;
#14861=CARTESIAN_POINT ( 'NONE',  ( 155.0000000000000568, -560.0000000000000000, -60.00000000000000711 ) ) ;
#14914=DIRECTION ( 'NONE',  ( 0.000000000000000000, 0.000000000000000000, 1.000000000000000000 ) ) ;
#14942=EDGE_CURVE ( 'NONE', #4421, #19824, #20442, .T. ) ;
#15009=LINE ( 'NONE', #18598, #5791 ) ;
#15052=VECTOR ( 'NONE', #4822, 1000.000000000000000 ) ;
#15091=CARTESIAN_POINT ( 'NONE',  ( 232.0000000000000284, 3.319562792410127342E-14, -56.99999999999973710 ) ) ;
#15182=DIRECTION ( 'NONE',  ( -1.000000000000000000, -2.775557561562891351E-17, 0.000000000000000000 ) ) ;
#15229=AXIS2_PLACEMENT_3D ( 'NONE', #1615, #7162, #10946 ) ;
#15243=ORIENTED_EDGE ( 'NONE', *, *, #1188, .F. ) ;
#15278=EDGE_CURVE ( 'NONE', #17629, #4760, #4276, .T. ) ;
#15304=CARTESIAN_POINT ( 'NONE',  ( 232.0000000000000568, -557.0000000000000000, 56.99999999999998579 ) ) ;
#15320=CARTESIAN_POINT ( 'NONE',  ( 158.0000000000000284, -500.0000000000000000, -29.99999999999997158 ) ) ;
#15384=CARTESIAN_POINT ( 'NONE',  ( 235.0000000000000284, -560.0000000000000000, -60.00000000000000711 ) ) ;
#15835=COLOUR_RGB ( '',0.8941176470588234615, 0.8941176470588234615, 0.8941176470588234615 ) ;
#15848=DIRECTION ( 'NONE',  ( 0.000000000000000000, -1.000000000000000000, -4.694093751100962712E-16 ) ) ;
#15871=ORIENTED_EDGE ( 'NONE', *, *, #1934, .T. ) ;
#16006=CARTESIAN_POINT ( 'NONE',  ( 158.0000000000000568, -557.0000000000000000, 0.000000000000000000 ) ) ;
#16041=AXIS2_PLACEMENT_3D ( 'NONE', #4580, #8326, #10274 ) ;
#16104=CARTESIAN_POINT ( 'NONE',  ( 155.0000000000000284, -489.9999999999998863, 60.00000000000000000 ) ) ;
#16122=DIRECTION ( 'NONE',  ( -2.775557561562891351E-17, 1.000000000000000000, 4.694093751100962712E-16 ) ) ;
#16198=DIRECTION ( 'NONE',  ( 1.302872740555339390E-32, -4.694093751100962712E-16, 1.000000000000000000 ) ) ;
#16201=FACE_OUTER_BOUND ( 'NONE', #3686, .T. ) ;
#16227=VECTOR ( 'NONE', #14137, 1000.000000000000000 ) ;
#16274=EDGE_CURVE ( 'NONE', #22960, #18604, #10958, .T. ) ;
#16284=LINE ( 'NONE', #7083, #6684 ) ;
#16378=CARTESIAN_POINT ( 'NONE',  ( 155.0000000000000284, -489.9999999999998863, 60.00000000000000000 ) ) ;
#16465=CYLINDRICAL_SURFACE ( 'NONE', #1510, 2.649999999999985700 ) ;
#16558=VECTOR ( 'NONE', #18784, 1000.000000000000000 ) ;
#16601=VECTOR ( 'NONE', #22247, 1000.000000000000000 ) ;
#16695=ORIENTED_EDGE ( 'NONE', *, *, #15278, .F. ) ;
#16751=CARTESIAN_POINT ( 'NONE',  ( 235.0000000000000284, -500.0000000000000000, 57.00000000000001421 ) ) ;
#16766=DIRECTION ( 'NONE',  ( 0.000000000000000000, -1.000000000000000000, -4.694093751100962712E-16 ) ) ;
#16779=VERTEX_POINT ( 'NONE', #16104 ) ;
#16791=CARTESIAN_POINT ( 'NONE',  ( 155.0000000000000284, -500.0000000000000000, 32.64999999999999858 ) ) ;
#16850=DIRECTION ( 'NONE',  ( 0.000000000000000000, 0.000000000000000000, -1.000000000000000000 ) ) ;
#16978=AXIS2_PLACEMENT_3D ( 'NONE', #18649, #17107, #11456 ) ;
#17066=DIRECTION ( 'NONE',  ( 0.000000000000000000, 0.000000000000000000, -1.000000000000000000 ) ) ;
#17078=DIRECTION ( 'NONE',  ( 0.000000000000000000, 0.000000000000000000, 1.000000000000000000 ) ) ;
#17107=DIRECTION ( 'NONE',  ( 1.000000000000000000, -0.000000000000000000, -0.000000000000000000 ) ) ;
#17135=CARTESIAN_POINT ( 'NONE',  ( 235.0000000000000284, -489.9999999999998863, 60.00000000000000000 ) ) ;
#17151=ORIENTED_EDGE ( 'NONE', *, *, #10037, .T. ) ;
#17257=ORIENTED_EDGE ( 'NONE', *, *, #9329, .T. ) ;
#17283=VERTEX_POINT ( 'NONE', #2864 ) ;
#17285=PLANE ( 'NONE',  #7985 ) ;
#17499=ORIENTED_EDGE ( 'NONE', *, *, #12955, .F. ) ;
#17598=CARTESIAN_POINT ( 'NONE',  ( 235.0000000000000284, -560.0000000000000000, 59.99999999999999289 ) ) ;
#17629=VERTEX_POINT ( 'NONE', #13375 ) ;
#17641=LINE ( 'NONE', #21506, #1280 ) ;
#17714=DIRECTION ( 'NONE',  ( 0.000000000000000000, 0.000000000000000000, -1.000000000000000000 ) ) ;
#17826=DIRECTION ( 'NONE',  ( 0.000000000000000000, 0.000000000000000000, 1.000000000000000000 ) ) ;
#17854=LINE ( 'NONE', #19300, #227 ) ;
#17873=DIRECTION ( 'NONE',  ( -1.000000000000000000, -2.775557561562891351E-17, 0.000000000000000000 ) ) ;
#17897=ORIENTED_EDGE ( 'NONE', *, *, #3148, .T. ) ;
#17968=ORIENTED_EDGE ( 'NONE', *, *, #12955, .T. ) ;
#17979=VECTOR ( 'NONE', #523, 1000.000000000000000 ) ;
#18037=VECTOR ( 'NONE', #6997, 1000.000000000000000 ) ;
#18051=VECTOR ( 'NONE', #4894, 1000.000000000000000 ) ;
#18057=EDGE_LOOP ( 'NONE', ( #11490, #4857 ) ) ;
#18125=DIRECTION ( 'NONE',  ( 1.000000000000000000, -0.000000000000000000, -0.000000000000000000 ) ) ;
#18198=ORIENTED_EDGE ( 'NONE', *, *, #21843, .T. ) ;
#18267=AXIS2_PLACEMENT_3D ( 'NONE', #8197, #22895, #17714 ) ;
#18340=PLANE ( 'NONE',  #13708 ) ;
#18366=ORIENTED_EDGE ( 'NONE', *, *, #21968, .T. ) ;
#18440=ORIENTED_EDGE ( 'NONE', *, *, #4149, .T. ) ;
#18458=APPLICATION_CONTEXT ( 'automotive_design' ) ;
#18463=EDGE_LOOP ( 'NONE', ( #17151, #20087, #16695, #12912 ) ) ;
#18530=CARTESIAN_POINT ( 'NONE',  ( 158.0000000000000284, -500.0000000000000000, -32.64999999999995595 ) ) ;
#18566=CARTESIAN_POINT ( 'NONE',  ( 158.0000000000000568, -557.0000000000000000, 56.99999999999998579 ) ) ;
#18584=ADVANCED_FACE ( 'NONE', ( #14236 ), #23377, .F. ) ;
#18586=( LENGTH_UNIT ( ) NAMED_UNIT ( * ) SI_UNIT ( .MILLI., .METRE. ) );
#18598=CARTESIAN_POINT ( 'NONE',  ( 158.0000000000000284, -490.0000000000000000, 9.066821367772113093E-13 ) ) ;
#18604=VERTEX_POINT ( 'NONE', #10130 ) ;
#18625=DIRECTION ( 'NONE',  ( -0.000000000000000000, 0.000000000000000000, 1.000000000000000000 ) ) ;
#18649=CARTESIAN_POINT ( 'NONE',  ( 158.0000000000000284, -500.0000000000000000, -29.99999999999997158 ) ) ;
#18715=ORIENTED_EDGE ( 'NONE', *, *, #10977, .F. ) ;
#18743=CARTESIAN_POINT ( 'NONE',  ( 158.0000000000000284, -500.0000000000000000, 27.35000000000002629 ) ) ;
#18784=DIRECTION ( 'NONE',  ( -2.775557561562891351E-17, 1.000000000000000000, 4.694093751100962712E-16 ) ) ;
#18785=ORIENTED_EDGE ( 'NONE', *, *, #9323, .T. ) ;
#18802=AXIS2_PLACEMENT_3D ( 'NONE', #6952, #19970, #5601 ) ;
#18818=CARTESIAN_POINT ( 'NONE',  ( 235.0000000000000284, -560.0000000000000000, 59.99999999999999289 ) ) ;
#18841=CIRCLE ( 'NONE', #14631, 2.649999999999985700 ) ;
#18868=ORIENTED_EDGE ( 'NONE', *, *, #320, .F. ) ;
#18888=CARTESIAN_POINT ( 'NONE',  ( 235.0000000000000284, -490.0000000000001137, -60.00000000000000000 ) ) ;
#19154=ORIENTED_EDGE ( 'NONE', *, *, #4589, .T. ) ;
#19155=VECTOR ( 'NONE', #5437, 1000.000000000000000 ) ;
#19204=ORIENTED_EDGE ( 'NONE', *, *, #8549, .T. ) ;
#19300=CARTESIAN_POINT ( 'NONE',  ( 158.0000000000000284, -500.0000000000000000, 32.64999999999999858 ) ) ;
#19305=EDGE_CURVE ( 'NONE', #9885, #14788, #2529, .T. ) ;
#19317=FACE_OUTER_BOUND ( 'NONE', #18463, .T. ) ;
#19331=EDGE_CURVE ( 'NONE', #9885, #18604, #718, .T. ) ;
#19339=SURFACE_STYLE_FILL_AREA ( #5102 ) ;
#19569=PRESENTATION_STYLE_ASSIGNMENT (( #8730 ) ) ;
#19581=VECTOR ( 'NONE', #6962, 1000.000000000000000 ) ;
#19824=VERTEX_POINT ( 'NONE', #23728 ) ;
#19842=ORIENTED_EDGE ( 'NONE', *, *, #12011, .T. ) ;
#19891=AXIS2_PLACEMENT_3D ( 'NONE', #22893, #23142, #6363 ) ;
#19962=FACE_OUTER_BOUND ( 'NONE', #12129, .T. ) ;
#19970=DIRECTION ( 'NONE',  ( -1.000000000000000000, -2.775557561562891351E-17, 0.000000000000000000 ) ) ;
#20025=EDGE_CURVE ( 'NONE', #20656, #12219, #2261, .T. ) ;
#20087=ORIENTED_EDGE ( 'NONE', *, *, #9156, .F. ) ;
#20163=ADVANCED_FACE ( 'NONE', ( #20191 ), #16465, .F. ) ;
#20191=FACE_OUTER_BOUND ( 'NONE', #21007, .T. ) ;
#20249=DIRECTION ( 'NONE',  ( -1.000000000000000000, -2.775557561562891351E-17, -0.000000000000000000 ) ) ;
#20252=VERTEX_POINT ( 'NONE', #638 ) ;
#20296=ORIENTED_EDGE ( 'NONE', *, *, #22469, .F. ) ;
#20422=VECTOR ( 'NONE', #610, 1000.000000000000000 ) ;
#20442=CIRCLE ( 'NONE', #16978, 2.649999999999985700 ) ;
#20487=LINE ( 'NONE', #15091, #16558 ) ;
#20633=VERTEX_POINT ( 'NONE', #16791 ) ;
#20656=VERTEX_POINT ( 'NONE', #2162 ) ;
#20759=CYLINDRICAL_SURFACE ( 'NONE', #3470, 2.649999999999985700 ) ;
#21007=EDGE_LOOP ( 'NONE', ( #10460, #10343, #19842, #18715 ) ) ;
#21128=DIRECTION ( 'NONE',  ( 5.135813185032629306E-32, -1.850371707708594366E-15, -1.000000000000000000 ) ) ;
#21138=VERTEX_POINT ( 'NONE', #15304 ) ;
#21289=( NAMED_UNIT ( * ) PLANE_ANGLE_UNIT ( ) SI_UNIT ( $, .RADIAN. ) );
#21363=CARTESIAN_POINT ( 'NONE',  ( 235.0000000000000284, -489.9999999999998863, 57.00000000000002132 ) ) ;
#21506=CARTESIAN_POINT ( 'NONE',  ( 235.0000000000000284, -490.0000000000001137, -56.99999999999996447 ) ) ;
#21542=DIRECTION ( 'NONE',  ( -1.000000000000000000, -2.775557561562891351E-17, 0.000000000000000000 ) ) ;
#21547=DIRECTION ( 'NONE',  ( 0.000000000000000000, 0.000000000000000000, 1.000000000000000000 ) ) ;
#21556=ORIENTED_EDGE ( 'NONE', *, *, #13297, .T. ) ;
#21635=VERTEX_POINT ( 'NONE', #12976 ) ;
#21703=ORIENTED_EDGE ( 'NONE', *, *, #5286, .F. ) ;
#21720=LINE ( 'NONE', #5178, #18037 ) ;
#21735=DIRECTION ( 'NONE',  ( -0.000000000000000000, 0.000000000000000000, 1.000000000000000000 ) ) ;
#21843=EDGE_CURVE ( 'NONE', #6345, #16779, #14729, .T. ) ;
#21899=VECTOR ( 'NONE', #14349, 1000.000000000000000 ) ;
#21968=EDGE_CURVE ( 'NONE', #8807, #6345, #21720, .T. ) ;
#22010=ORIENTED_EDGE ( 'NONE', *, *, #4149, .F. ) ;
#22029=CARTESIAN_POINT ( 'NONE',  ( 158.0000000000000284, -2.237095343400623696E-14, 57.00000000000024869 ) ) ;
#22062=EDGE_LOOP ( 'NONE', ( #22790, #5533 ) ) ;
#22247=DIRECTION ( 'NONE',  ( -2.775557561562891351E-17, 1.000000000000000000, -2.081668171172166936E-15 ) ) ;
#22263=ADVANCED_FACE ( 'NONE', ( #4526 ), #5980, .T. ) ;
#22284=ORIENTED_EDGE ( 'NONE', *, *, #19331, .F. ) ;
#22405=PLANE ( 'NONE',  #9222 ) ;
#22415=DIRECTION ( 'NONE',  ( -1.000000000000000000, -2.775557561562891351E-17, 0.000000000000000000 ) ) ;
#22458=DIRECTION ( 'NONE',  ( -1.000000000000000000, -2.775557561562891351E-17, 0.000000000000000000 ) ) ;
#22469=EDGE_CURVE ( 'NONE', #11416, #10663, #2987, .T. ) ;
#22660=UNCERTAINTY_MEASURE_WITH_UNIT (LENGTH_MEASURE( 1.000000000000000082E-05 ), #3030, 'distance_accuracy_value', 'NONE');
#22662=AXIS2_PLACEMENT_3D ( 'NONE', #13389, #13524, #8040 ) ;
#22698=CIRCLE ( 'NONE', #14637, 2.650000000000041211 ) ;
#22735=ORIENTED_EDGE ( 'NONE', *, *, #6445, .F. ) ;
#22790=ORIENTED_EDGE ( 'NONE', *, *, #20025, .F. ) ;
#22802=FACE_OUTER_BOUND ( 'NONE', #12091, .T. ) ;
#22884=CARTESIAN_POINT ( 'NONE',  ( 158.0000000000000568, -557.0000000000000000, -57.00000000000000000 ) ) ;
#22893=CARTESIAN_POINT ( 'NONE',  ( 158.0000000000000284, -500.0000000000000000, 30.00000000000001421 ) ) ;
#22895=DIRECTION ( 'NONE',  ( 1.000000000000000000, -0.000000000000000000, -0.000000000000000000 ) ) ;
#22943=EDGE_LOOP ( 'NONE', ( #9311, #6530, #11705, #21556 ) ) ;
#22960=VERTEX_POINT ( 'NONE', #18566 ) ;
#22991=ADVANCED_FACE ( 'NONE', ( #9409 ), #13419, .T. ) ;
#23043=EDGE_LOOP ( 'NONE', ( #22735, #20296 ) ) ;
#23142=DIRECTION ( 'NONE',  ( 1.000000000000000000, -0.000000000000000000, -0.000000000000000000 ) ) ;
#23143=LINE ( 'NONE', #16378, #4639 ) ;
#23245=LINE ( 'NONE', #13769, #5720 ) ;
#23255=APPLICATION_CONTEXT ( 'automotive_design' ) ;
#23324=( NAMED_UNIT ( * ) SI_UNIT ( $, .STERADIAN. ) SOLID_ANGLE_UNIT ( ) );
#23377=CYLINDRICAL_SURFACE ( 'NONE', #19891, 2.649999999999985700 ) ;
#23410=ORIENTED_EDGE ( 'NONE', *, *, #19305, .F. ) ;
#23443=ADVANCED_FACE ( 'NONE', ( #9915 ), #22405, .T. ) ;
#23483=EDGE_LOOP ( 'NONE', ( #2871, #22284, #6275, #18440 ) ) ;
#23666=PRODUCT ( 'bucket', 'bucket', '', ( #3706 ) ) ;
#23728=CARTESIAN_POINT ( 'NONE',  ( 158.0000000000000284, -500.0000000000000000, -27.34999999999998721 ) ) ;
#23741=CARTESIAN_POINT ( 'NONE',  ( 232.0000000000000284, -490.0000000000001137, -56.99999999999996447 ) ) ;
#23907=COLOUR_RGB('Sky Blue',0.24,0.69,0.87);
#23908=FILL_AREA_STYLE_COLOUR('',#23907);
#23909=FILL_AREA_STYLE('',(#23908));
#23910=SURFACE_STYLE_FILL_AREA(#23909);
#23911=SURFACE_SIDE_STYLE('',(#23910));
#23912=SURFACE_STYLE_USAGE(.BOTH.,#23911);
#23913=PRESENTATION_STYLE_ASSIGNMENT((#23912));
ENDSEC;
END-ISO-10303-21;
